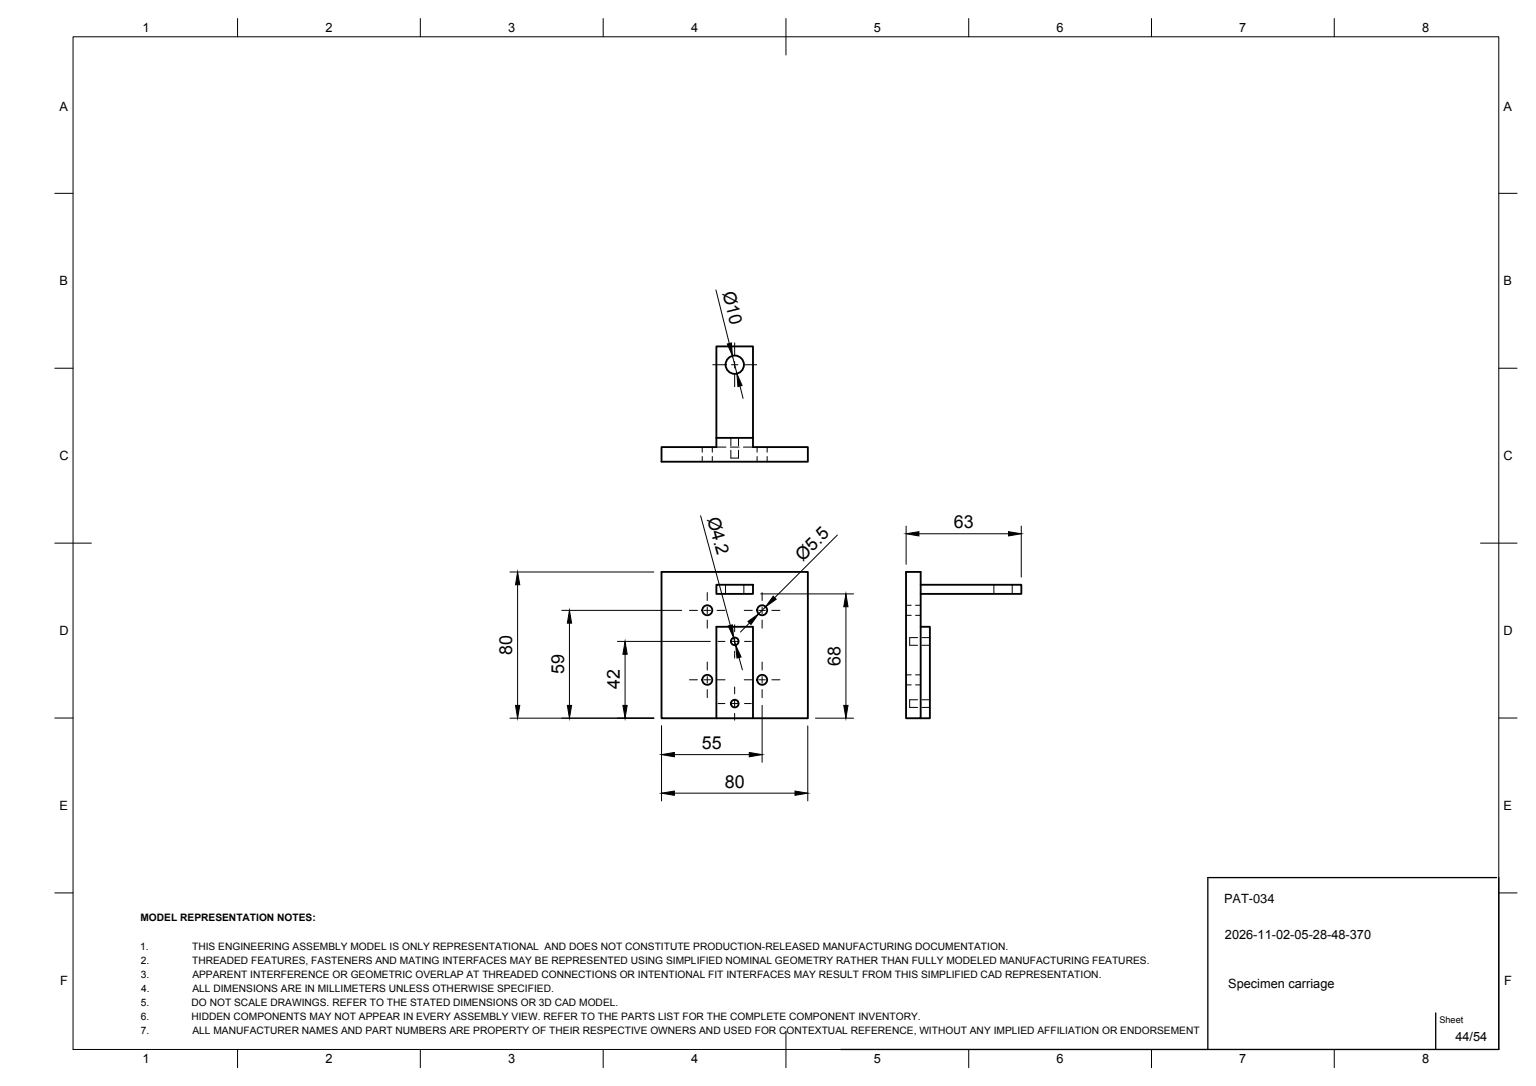
ISO-10303-21;
HEADER;
/* Generated by software containing ST-Developer
 * from STEP Tools, Inc. (www.steptools.com) 
 */

FILE_DESCRIPTION(
/* description */ ('Fatigue rig crank-slider'),
/* implementation_level */ '2;1');

FILE_NAME(
/* name */ 'Specimen carriage.step',
/* time_stamp */ '2026-10-28T03:24:50-07:00',
/* author */ (''),
/* organization */ (''),
/* preprocessor_version */ 'ST-DEVELOPER v20.2',
/* originating_system */ 'Autodesk Translation Framework v15.17.0.0',
/* authorisation */ '');

FILE_SCHEMA (('AUTOMOTIVE_DESIGN { 1 0 10303 214 3 1 1 }'));
ENDSEC;

DATA;
#10=MECHANICAL_DESIGN_GEOMETRIC_PRESENTATION_REPRESENTATION('',(#633),#16911);
#524=SHAPE_REPRESENTATION_RELATIONSHIP('SRR','None',#17168,#574);
#574=ADVANCED_BREP_SHAPE_REPRESENTATION('',(#690),#16897);
#633=STYLED_ITEM('',(#17501),#690);
#690=MANIFOLD_SOLID_BREP('Body1',#8926);
#863=FACE_BOUND('',#2286,.T.);
#864=FACE_BOUND('',#2287,.T.);
#865=FACE_BOUND('',#2291,.T.);
#866=FACE_BOUND('',#2296,.T.);
#867=FACE_BOUND('',#2306,.T.);
#868=FACE_BOUND('',#2307,.T.);
#869=FACE_BOUND('',#2308,.T.);
#870=FACE_BOUND('',#2309,.T.);
#871=FACE_BOUND('',#2310,.T.);
#872=FACE_BOUND('',#2312,.T.);
#873=FACE_BOUND('',#2313,.T.);
#874=FACE_BOUND('',#2314,.T.);
#875=FACE_BOUND('',#2315,.T.);
#1111=PLANE('',#10252);
#1112=PLANE('',#10256);
#1113=PLANE('',#10257);
#1114=PLANE('',#10258);
#1115=PLANE('',#10259);
#1116=PLANE('',#10260);
#1117=PLANE('',#10264);
#1118=PLANE('',#10265);
#1119=PLANE('',#10266);
#1120=PLANE('',#10267);
#1121=PLANE('',#10268);
#1122=PLANE('',#10281);
#1123=PLANE('',#10282);
#1124=PLANE('',#10283);
#1125=PLANE('',#10284);
#1126=PLANE('',#10285);
#1127=PLANE('',#10286);
#1593=FACE_OUTER_BOUND('',#2279,.T.);
#1594=FACE_OUTER_BOUND('',#2280,.T.);
#1595=FACE_OUTER_BOUND('',#2281,.T.);
#1596=FACE_OUTER_BOUND('',#2282,.T.);
#1597=FACE_OUTER_BOUND('',#2283,.T.);
#1598=FACE_OUTER_BOUND('',#2284,.T.);
#1599=FACE_OUTER_BOUND('',#2285,.T.);
#1600=FACE_OUTER_BOUND('',#2288,.T.);
#1601=FACE_OUTER_BOUND('',#2289,.T.);
#1602=FACE_OUTER_BOUND('',#2290,.T.);
#1603=FACE_OUTER_BOUND('',#2292,.T.);
#1604=FACE_OUTER_BOUND('',#2293,.T.);
#1605=FACE_OUTER_BOUND('',#2294,.T.);
#1606=FACE_OUTER_BOUND('',#2295,.T.);
#1607=FACE_OUTER_BOUND('',#2297,.T.);
#1608=FACE_OUTER_BOUND('',#2298,.T.);
#1609=FACE_OUTER_BOUND('',#2299,.T.);
#1610=FACE_OUTER_BOUND('',#2300,.T.);
#1611=FACE_OUTER_BOUND('',#2301,.T.);
#1612=FACE_OUTER_BOUND('',#2302,.T.);
#1613=FACE_OUTER_BOUND('',#2303,.T.);
#1614=FACE_OUTER_BOUND('',#2304,.T.);
#1615=FACE_OUTER_BOUND('',#2305,.T.);
#1616=FACE_OUTER_BOUND('',#2311,.T.);
#2279=EDGE_LOOP('',(#7552,#7553,#7554,#7555));
#2280=EDGE_LOOP('',(#7556));
#2281=EDGE_LOOP('',(#7557,#7558,#7559,#7560));
#2282=EDGE_LOOP('',(#7561));
#2283=EDGE_LOOP('',(#7562,#7563,#7564,#7565));
#2284=EDGE_LOOP('',(#7566,#7567,#7568,#7569));
#2285=EDGE_LOOP('',(#7570,#7571,#7572,#7573));
#2286=EDGE_LOOP('',(#7574));
#2287=EDGE_LOOP('',(#7575));
#2288=EDGE_LOOP('',(#7576,#7577,#7578,#7579));
#2289=EDGE_LOOP('',(#7580,#7581,#7582,#7583));
#2290=EDGE_LOOP('',(#7584,#7585,#7586,#7587));
#2291=EDGE_LOOP('',(#7588));
#2292=EDGE_LOOP('',(#7589,#7590,#7591,#7592));
#2293=EDGE_LOOP('',(#7593,#7594,#7595,#7596));
#2294=EDGE_LOOP('',(#7597,#7598,#7599,#7600));
#2295=EDGE_LOOP('',(#7601,#7602,#7603,#7604));
#2296=EDGE_LOOP('',(#7605));
#2297=EDGE_LOOP('',(#7606,#7607,#7608,#7609));
#2298=EDGE_LOOP('',(#7610,#7611,#7612,#7613));
#2299=EDGE_LOOP('',(#7614,#7615,#7616,#7617));
#2300=EDGE_LOOP('',(#7618,#7619,#7620,#7621));
#2301=EDGE_LOOP('',(#7622,#7623,#7624,#7625));
#2302=EDGE_LOOP('',(#7626,#7627,#7628,#7629));
#2303=EDGE_LOOP('',(#7630,#7631,#7632,#7633,#7634,#7635,#7636,#7637));
#2304=EDGE_LOOP('',(#7638,#7639,#7640,#7641));
#2305=EDGE_LOOP('',(#7642,#7643,#7644,#7645,#7646,#7647,#7648,#7649));
#2306=EDGE_LOOP('',(#7650,#7651,#7652,#7653));
#2307=EDGE_LOOP('',(#7654));
#2308=EDGE_LOOP('',(#7655));
#2309=EDGE_LOOP('',(#7656));
#2310=EDGE_LOOP('',(#7657));
#2311=EDGE_LOOP('',(#7658,#7659,#7660,#7661));
#2312=EDGE_LOOP('',(#7662));
#2313=EDGE_LOOP('',(#7663));
#2314=EDGE_LOOP('',(#7664));
#2315=EDGE_LOOP('',(#7665));
#2863=LINE('',#16027,#3509);
#2864=LINE('',#16034,#3510);
#2865=LINE('',#16040,#3511);
#2866=LINE('',#16042,#3512);
#2867=LINE('',#16044,#3513);
#2868=LINE('',#16045,#3514);
#2869=LINE('',#16049,#3515);
#2870=LINE('',#16051,#3516);
#2871=LINE('',#16053,#3517);
#2872=LINE('',#16054,#3518);
#2873=LINE('',#16056,#3519);
#2874=LINE('',#16057,#3520);
#2875=LINE('',#16059,#3521);
#2876=LINE('',#16064,#3522);
#2877=LINE('',#16069,#3523);
#2878=LINE('',#16071,#3524);
#2879=LINE('',#16073,#3525);
#2880=LINE('',#16074,#3526);
#2881=LINE('',#16077,#3527);
#2882=LINE('',#16079,#3528);
#2883=LINE('',#16080,#3529);
#2884=LINE('',#16083,#3530);
#2885=LINE('',#16085,#3531);
#2886=LINE('',#16086,#3532);
#2887=LINE('',#16088,#3533);
#2888=LINE('',#16090,#3534);
#2889=LINE('',#16095,#3535);
#2890=LINE('',#16101,#3536);
#2891=LINE('',#16107,#3537);
#2892=LINE('',#16113,#3538);
#2893=LINE('',#16118,#3539);
#2894=LINE('',#16120,#3540);
#2895=LINE('',#16122,#3541);
#2896=LINE('',#16123,#3542);
#2897=LINE('',#16126,#3543);
#2898=LINE('',#16128,#3544);
#2899=LINE('',#16129,#3545);
#2900=LINE('',#16132,#3546);
#2901=LINE('',#16133,#3547);
#2902=LINE('',#16135,#3548);
#2903=LINE('',#16136,#3549);
#2904=LINE('',#16138,#3550);
#2905=LINE('',#16139,#3551);
#3509=VECTOR('',#12485,0.210000000000001);
#3510=VECTOR('',#12494,0.210000000000001);
#3511=VECTOR('',#12501,1.);
#3512=VECTOR('',#12502,1.);
#3513=VECTOR('',#12503,1.);
#3514=VECTOR('',#12504,1.);
#3515=VECTOR('',#12507,1.);
#3516=VECTOR('',#12508,1.);
#3517=VECTOR('',#12509,1.);
#3518=VECTOR('',#12510,1.);
#3519=VECTOR('',#12513,1.);
#3520=VECTOR('',#12514,1.);
#3521=VECTOR('',#12517,1.);
#3522=VECTOR('',#12522,0.5);
#3523=VECTOR('',#12527,1.);
#3524=VECTOR('',#12528,1.);
#3525=VECTOR('',#12529,1.);
#3526=VECTOR('',#12530,1.);
#3527=VECTOR('',#12533,1.);
#3528=VECTOR('',#12534,1.);
#3529=VECTOR('',#12535,1.);
#3530=VECTOR('',#12538,1.);
#3531=VECTOR('',#12539,1.);
#3532=VECTOR('',#12540,1.);
#3533=VECTOR('',#12543,1.);
#3534=VECTOR('',#12546,1.);
#3535=VECTOR('',#12551,0.275);
#3536=VECTOR('',#12558,0.275);
#3537=VECTOR('',#12565,0.275);
#3538=VECTOR('',#12572,0.275);
#3539=VECTOR('',#12577,1.);
#3540=VECTOR('',#12578,1.);
#3541=VECTOR('',#12579,1.);
#3542=VECTOR('',#12580,1.);
#3543=VECTOR('',#12583,1.);
#3544=VECTOR('',#12584,1.);
#3545=VECTOR('',#12585,1.);
#3546=VECTOR('',#12588,1.);
#3547=VECTOR('',#12589,1.);
#3548=VECTOR('',#12590,1.);
#3549=VECTOR('',#12591,1.);
#3550=VECTOR('',#12594,1.);
#3551=VECTOR('',#12595,1.);
#4073=CIRCLE('',#10250,0.210000000000001);
#4074=CIRCLE('',#10251,0.210000000000001);
#4075=CIRCLE('',#10254,0.210000000000001);
#4076=CIRCLE('',#10255,0.210000000000001);
#4077=CIRCLE('',#10262,0.5);
#4078=CIRCLE('',#10263,0.5);
#4079=CIRCLE('',#10270,0.275);
#4080=CIRCLE('',#10271,0.275);
#4081=CIRCLE('',#10273,0.275);
#4082=CIRCLE('',#10274,0.275);
#4083=CIRCLE('',#10276,0.275);
#4084=CIRCLE('',#10277,0.275);
#4085=CIRCLE('',#10279,0.275);
#4086=CIRCLE('',#10280,0.275);
#4685=VERTEX_POINT('',#16024);
#4686=VERTEX_POINT('',#16026);
#4687=VERTEX_POINT('',#16031);
#4688=VERTEX_POINT('',#16033);
#4689=VERTEX_POINT('',#16038);
#4690=VERTEX_POINT('',#16039);
#4691=VERTEX_POINT('',#16041);
#4692=VERTEX_POINT('',#16043);
#4693=VERTEX_POINT('',#16047);
#4694=VERTEX_POINT('',#16048);
#4695=VERTEX_POINT('',#16050);
#4696=VERTEX_POINT('',#16052);
#4697=VERTEX_POINT('',#16061);
#4698=VERTEX_POINT('',#16063);
#4699=VERTEX_POINT('',#16067);
#4700=VERTEX_POINT('',#16068);
#4701=VERTEX_POINT('',#16070);
#4702=VERTEX_POINT('',#16072);
#4703=VERTEX_POINT('',#16076);
#4704=VERTEX_POINT('',#16078);
#4705=VERTEX_POINT('',#16082);
#4706=VERTEX_POINT('',#16084);
#4707=VERTEX_POINT('',#16092);
#4708=VERTEX_POINT('',#16094);
#4709=VERTEX_POINT('',#16098);
#4710=VERTEX_POINT('',#16100);
#4711=VERTEX_POINT('',#16104);
#4712=VERTEX_POINT('',#16106);
#4713=VERTEX_POINT('',#16110);
#4714=VERTEX_POINT('',#16112);
#4715=VERTEX_POINT('',#16116);
#4716=VERTEX_POINT('',#16117);
#4717=VERTEX_POINT('',#16119);
#4718=VERTEX_POINT('',#16121);
#4719=VERTEX_POINT('',#16125);
#4720=VERTEX_POINT('',#16127);
#4721=VERTEX_POINT('',#16131);
#4722=VERTEX_POINT('',#16134);
#5674=EDGE_CURVE('',#4685,#4685,#4073,.T.);
#5675=EDGE_CURVE('',#4685,#4686,#2863,.T.);
#5676=EDGE_CURVE('',#4686,#4686,#4074,.T.);
#5677=EDGE_CURVE('',#4687,#4687,#4075,.T.);
#5678=EDGE_CURVE('',#4687,#4688,#2864,.T.);
#5679=EDGE_CURVE('',#4688,#4688,#4076,.T.);
#5680=EDGE_CURVE('',#4689,#4690,#2865,.T.);
#5681=EDGE_CURVE('',#4689,#4691,#2866,.T.);
#5682=EDGE_CURVE('',#4692,#4691,#2867,.T.);
#5683=EDGE_CURVE('',#4690,#4692,#2868,.T.);
#5684=EDGE_CURVE('',#4693,#4694,#2869,.T.);
#5685=EDGE_CURVE('',#4695,#4693,#2870,.T.);
#5686=EDGE_CURVE('',#4696,#4695,#2871,.T.);
#5687=EDGE_CURVE('',#4694,#4696,#2872,.T.);
#5688=EDGE_CURVE('',#4694,#4689,#2873,.T.);
#5689=EDGE_CURVE('',#4691,#4696,#2874,.T.);
#5690=EDGE_CURVE('',#4692,#4695,#2875,.T.);
#5691=EDGE_CURVE('',#4697,#4697,#4077,.T.);
#5692=EDGE_CURVE('',#4697,#4698,#2876,.T.);
#5693=EDGE_CURVE('',#4698,#4698,#4078,.T.);
#5694=EDGE_CURVE('',#4699,#4700,#2877,.T.);
#5695=EDGE_CURVE('',#4699,#4701,#2878,.T.);
#5696=EDGE_CURVE('',#4701,#4702,#2879,.T.);
#5697=EDGE_CURVE('',#4702,#4700,#2880,.T.);
#5698=EDGE_CURVE('',#4703,#4699,#2881,.T.);
#5699=EDGE_CURVE('',#4704,#4703,#2882,.T.);
#5700=EDGE_CURVE('',#4701,#4704,#2883,.T.);
#5701=EDGE_CURVE('',#4700,#4705,#2884,.T.);
#5702=EDGE_CURVE('',#4702,#4706,#2885,.T.);
#5703=EDGE_CURVE('',#4705,#4706,#2886,.T.);
#5704=EDGE_CURVE('',#4706,#4704,#2887,.T.);
#5705=EDGE_CURVE('',#4705,#4703,#2888,.T.);
#5706=EDGE_CURVE('',#4707,#4707,#4079,.T.);
#5707=EDGE_CURVE('',#4707,#4708,#2889,.T.);
#5708=EDGE_CURVE('',#4708,#4708,#4080,.T.);
#5709=EDGE_CURVE('',#4709,#4709,#4081,.T.);
#5710=EDGE_CURVE('',#4709,#4710,#2890,.T.);
#5711=EDGE_CURVE('',#4710,#4710,#4082,.T.);
#5712=EDGE_CURVE('',#4711,#4711,#4083,.T.);
#5713=EDGE_CURVE('',#4711,#4712,#2891,.T.);
#5714=EDGE_CURVE('',#4712,#4712,#4084,.T.);
#5715=EDGE_CURVE('',#4713,#4713,#4085,.T.);
#5716=EDGE_CURVE('',#4713,#4714,#2892,.T.);
#5717=EDGE_CURVE('',#4714,#4714,#4086,.T.);
#5718=EDGE_CURVE('',#4715,#4716,#2893,.T.);
#5719=EDGE_CURVE('',#4716,#4717,#2894,.T.);
#5720=EDGE_CURVE('',#4718,#4717,#2895,.T.);
#5721=EDGE_CURVE('',#4715,#4718,#2896,.T.);
#5722=EDGE_CURVE('',#4719,#4715,#2897,.T.);
#5723=EDGE_CURVE('',#4720,#4718,#2898,.T.);
#5724=EDGE_CURVE('',#4719,#4720,#2899,.T.);
#5725=EDGE_CURVE('',#4721,#4719,#2900,.T.);
#5726=EDGE_CURVE('',#4693,#4720,#2901,.T.);
#5727=EDGE_CURVE('',#4722,#4690,#2902,.T.);
#5728=EDGE_CURVE('',#4721,#4722,#2903,.T.);
#5729=EDGE_CURVE('',#4716,#4721,#2904,.T.);
#5730=EDGE_CURVE('',#4717,#4722,#2905,.T.);
#7552=ORIENTED_EDGE('',*,*,#5674,.F.);
#7553=ORIENTED_EDGE('',*,*,#5675,.T.);
#7554=ORIENTED_EDGE('',*,*,#5676,.F.);
#7555=ORIENTED_EDGE('',*,*,#5675,.F.);
#7556=ORIENTED_EDGE('',*,*,#5674,.T.);
#7557=ORIENTED_EDGE('',*,*,#5677,.F.);
#7558=ORIENTED_EDGE('',*,*,#5678,.T.);
#7559=ORIENTED_EDGE('',*,*,#5679,.F.);
#7560=ORIENTED_EDGE('',*,*,#5678,.F.);
#7561=ORIENTED_EDGE('',*,*,#5677,.T.);
#7562=ORIENTED_EDGE('',*,*,#5680,.F.);
#7563=ORIENTED_EDGE('',*,*,#5681,.T.);
#7564=ORIENTED_EDGE('',*,*,#5682,.F.);
#7565=ORIENTED_EDGE('',*,*,#5683,.F.);
#7566=ORIENTED_EDGE('',*,*,#5684,.F.);
#7567=ORIENTED_EDGE('',*,*,#5685,.F.);
#7568=ORIENTED_EDGE('',*,*,#5686,.F.);
#7569=ORIENTED_EDGE('',*,*,#5687,.F.);
#7570=ORIENTED_EDGE('',*,*,#5688,.F.);
#7571=ORIENTED_EDGE('',*,*,#5687,.T.);
#7572=ORIENTED_EDGE('',*,*,#5689,.F.);
#7573=ORIENTED_EDGE('',*,*,#5681,.F.);
#7574=ORIENTED_EDGE('',*,*,#5676,.T.);
#7575=ORIENTED_EDGE('',*,*,#5679,.T.);
#7576=ORIENTED_EDGE('',*,*,#5689,.T.);
#7577=ORIENTED_EDGE('',*,*,#5686,.T.);
#7578=ORIENTED_EDGE('',*,*,#5690,.F.);
#7579=ORIENTED_EDGE('',*,*,#5682,.T.);
#7580=ORIENTED_EDGE('',*,*,#5691,.F.);
#7581=ORIENTED_EDGE('',*,*,#5692,.T.);
#7582=ORIENTED_EDGE('',*,*,#5693,.F.);
#7583=ORIENTED_EDGE('',*,*,#5692,.F.);
#7584=ORIENTED_EDGE('',*,*,#5694,.F.);
#7585=ORIENTED_EDGE('',*,*,#5695,.T.);
#7586=ORIENTED_EDGE('',*,*,#5696,.T.);
#7587=ORIENTED_EDGE('',*,*,#5697,.T.);
#7588=ORIENTED_EDGE('',*,*,#5691,.T.);
#7589=ORIENTED_EDGE('',*,*,#5698,.F.);
#7590=ORIENTED_EDGE('',*,*,#5699,.F.);
#7591=ORIENTED_EDGE('',*,*,#5700,.F.);
#7592=ORIENTED_EDGE('',*,*,#5695,.F.);
#7593=ORIENTED_EDGE('',*,*,#5701,.F.);
#7594=ORIENTED_EDGE('',*,*,#5697,.F.);
#7595=ORIENTED_EDGE('',*,*,#5702,.T.);
#7596=ORIENTED_EDGE('',*,*,#5703,.F.);
#7597=ORIENTED_EDGE('',*,*,#5696,.F.);
#7598=ORIENTED_EDGE('',*,*,#5700,.T.);
#7599=ORIENTED_EDGE('',*,*,#5704,.F.);
#7600=ORIENTED_EDGE('',*,*,#5702,.F.);
#7601=ORIENTED_EDGE('',*,*,#5705,.F.);
#7602=ORIENTED_EDGE('',*,*,#5703,.T.);
#7603=ORIENTED_EDGE('',*,*,#5704,.T.);
#7604=ORIENTED_EDGE('',*,*,#5699,.T.);
#7605=ORIENTED_EDGE('',*,*,#5693,.T.);
#7606=ORIENTED_EDGE('',*,*,#5706,.F.);
#7607=ORIENTED_EDGE('',*,*,#5707,.T.);
#7608=ORIENTED_EDGE('',*,*,#5708,.F.);
#7609=ORIENTED_EDGE('',*,*,#5707,.F.);
#7610=ORIENTED_EDGE('',*,*,#5709,.F.);
#7611=ORIENTED_EDGE('',*,*,#5710,.T.);
#7612=ORIENTED_EDGE('',*,*,#5711,.F.);
#7613=ORIENTED_EDGE('',*,*,#5710,.F.);
#7614=ORIENTED_EDGE('',*,*,#5712,.F.);
#7615=ORIENTED_EDGE('',*,*,#5713,.T.);
#7616=ORIENTED_EDGE('',*,*,#5714,.F.);
#7617=ORIENTED_EDGE('',*,*,#5713,.F.);
#7618=ORIENTED_EDGE('',*,*,#5715,.F.);
#7619=ORIENTED_EDGE('',*,*,#5716,.T.);
#7620=ORIENTED_EDGE('',*,*,#5717,.F.);
#7621=ORIENTED_EDGE('',*,*,#5716,.F.);
#7622=ORIENTED_EDGE('',*,*,#5718,.T.);
#7623=ORIENTED_EDGE('',*,*,#5719,.T.);
#7624=ORIENTED_EDGE('',*,*,#5720,.F.);
#7625=ORIENTED_EDGE('',*,*,#5721,.F.);
#7626=ORIENTED_EDGE('',*,*,#5722,.T.);
#7627=ORIENTED_EDGE('',*,*,#5721,.T.);
#7628=ORIENTED_EDGE('',*,*,#5723,.F.);
#7629=ORIENTED_EDGE('',*,*,#5724,.F.);
#7630=ORIENTED_EDGE('',*,*,#5725,.T.);
#7631=ORIENTED_EDGE('',*,*,#5724,.T.);
#7632=ORIENTED_EDGE('',*,*,#5726,.F.);
#7633=ORIENTED_EDGE('',*,*,#5684,.T.);
#7634=ORIENTED_EDGE('',*,*,#5688,.T.);
#7635=ORIENTED_EDGE('',*,*,#5680,.T.);
#7636=ORIENTED_EDGE('',*,*,#5727,.F.);
#7637=ORIENTED_EDGE('',*,*,#5728,.F.);
#7638=ORIENTED_EDGE('',*,*,#5729,.T.);
#7639=ORIENTED_EDGE('',*,*,#5728,.T.);
#7640=ORIENTED_EDGE('',*,*,#5730,.F.);
#7641=ORIENTED_EDGE('',*,*,#5719,.F.);
#7642=ORIENTED_EDGE('',*,*,#5685,.T.);
#7643=ORIENTED_EDGE('',*,*,#5726,.T.);
#7644=ORIENTED_EDGE('',*,*,#5723,.T.);
#7645=ORIENTED_EDGE('',*,*,#5720,.T.);
#7646=ORIENTED_EDGE('',*,*,#5730,.T.);
#7647=ORIENTED_EDGE('',*,*,#5727,.T.);
#7648=ORIENTED_EDGE('',*,*,#5683,.T.);
#7649=ORIENTED_EDGE('',*,*,#5690,.T.);
#7650=ORIENTED_EDGE('',*,*,#5698,.T.);
#7651=ORIENTED_EDGE('',*,*,#5694,.T.);
#7652=ORIENTED_EDGE('',*,*,#5701,.T.);
#7653=ORIENTED_EDGE('',*,*,#5705,.T.);
#7654=ORIENTED_EDGE('',*,*,#5708,.T.);
#7655=ORIENTED_EDGE('',*,*,#5711,.T.);
#7656=ORIENTED_EDGE('',*,*,#5714,.T.);
#7657=ORIENTED_EDGE('',*,*,#5717,.T.);
#7658=ORIENTED_EDGE('',*,*,#5729,.F.);
#7659=ORIENTED_EDGE('',*,*,#5718,.F.);
#7660=ORIENTED_EDGE('',*,*,#5722,.F.);
#7661=ORIENTED_EDGE('',*,*,#5725,.F.);
#7662=ORIENTED_EDGE('',*,*,#5706,.T.);
#7663=ORIENTED_EDGE('',*,*,#5709,.T.);
#7664=ORIENTED_EDGE('',*,*,#5712,.T.);
#7665=ORIENTED_EDGE('',*,*,#5715,.T.);
#8325=CYLINDRICAL_SURFACE('',#10249,0.210000000000001);
#8326=CYLINDRICAL_SURFACE('',#10253,0.210000000000001);
#8327=CYLINDRICAL_SURFACE('',#10261,0.5);
#8328=CYLINDRICAL_SURFACE('',#10269,0.275);
#8329=CYLINDRICAL_SURFACE('',#10272,0.275);
#8330=CYLINDRICAL_SURFACE('',#10275,0.275);
#8331=CYLINDRICAL_SURFACE('',#10278,0.275);
#8731=ADVANCED_FACE('',(#1593),#8325,.F.);
#8732=ADVANCED_FACE('',(#1594),#1111,.T.);
#8733=ADVANCED_FACE('',(#1595),#8326,.F.);
#8734=ADVANCED_FACE('',(#1596),#1112,.T.);
#8735=ADVANCED_FACE('',(#1597),#1113,.T.);
#8736=ADVANCED_FACE('',(#1598),#1114,.T.);
#8737=ADVANCED_FACE('',(#1599,#863,#864),#1115,.T.);
#8738=ADVANCED_FACE('',(#1600),#1116,.T.);
#8739=ADVANCED_FACE('',(#1601),#8327,.F.);
#8740=ADVANCED_FACE('',(#1602,#865),#1117,.F.);
#8741=ADVANCED_FACE('',(#1603),#1118,.T.);
#8742=ADVANCED_FACE('',(#1604),#1119,.T.);
#8743=ADVANCED_FACE('',(#1605),#1120,.T.);
#8744=ADVANCED_FACE('',(#1606,#866),#1121,.T.);
#8745=ADVANCED_FACE('',(#1607),#8328,.F.);
#8746=ADVANCED_FACE('',(#1608),#8329,.F.);
#8747=ADVANCED_FACE('',(#1609),#8330,.F.);
#8748=ADVANCED_FACE('',(#1610),#8331,.F.);
#8749=ADVANCED_FACE('',(#1611),#1122,.T.);
#8750=ADVANCED_FACE('',(#1612),#1123,.T.);
#8751=ADVANCED_FACE('',(#1613),#1124,.T.);
#8752=ADVANCED_FACE('',(#1614),#1125,.T.);
#8753=ADVANCED_FACE('',(#1615,#867,#868,#869,#870,#871),#1126,.T.);
#8754=ADVANCED_FACE('',(#1616,#872,#873,#874,#875),#1127,.F.);
#8926=CLOSED_SHELL('',(#8731,#8732,#8733,#8734,#8735,#8736,#8737,#8738,
#8739,#8740,#8741,#8742,#8743,#8744,#8745,#8746,#8747,#8748,#8749,#8750,
#8751,#8752,#8753,#8754));
#10248=AXIS2_PLACEMENT_3D('',#16022,#12479,#12480);
#10249=AXIS2_PLACEMENT_3D('',#16023,#12481,#12482);
#10250=AXIS2_PLACEMENT_3D('',#16025,#12483,#12484);
#10251=AXIS2_PLACEMENT_3D('',#16028,#12486,#12487);
#10252=AXIS2_PLACEMENT_3D('',#16029,#12488,#12489);
#10253=AXIS2_PLACEMENT_3D('',#16030,#12490,#12491);
#10254=AXIS2_PLACEMENT_3D('',#16032,#12492,#12493);
#10255=AXIS2_PLACEMENT_3D('',#16035,#12495,#12496);
#10256=AXIS2_PLACEMENT_3D('',#16036,#12497,#12498);
#10257=AXIS2_PLACEMENT_3D('',#16037,#12499,#12500);
#10258=AXIS2_PLACEMENT_3D('',#16046,#12505,#12506);
#10259=AXIS2_PLACEMENT_3D('',#16055,#12511,#12512);
#10260=AXIS2_PLACEMENT_3D('',#16058,#12515,#12516);
#10261=AXIS2_PLACEMENT_3D('',#16060,#12518,#12519);
#10262=AXIS2_PLACEMENT_3D('',#16062,#12520,#12521);
#10263=AXIS2_PLACEMENT_3D('',#16065,#12523,#12524);
#10264=AXIS2_PLACEMENT_3D('',#16066,#12525,#12526);
#10265=AXIS2_PLACEMENT_3D('',#16075,#12531,#12532);
#10266=AXIS2_PLACEMENT_3D('',#16081,#12536,#12537);
#10267=AXIS2_PLACEMENT_3D('',#16087,#12541,#12542);
#10268=AXIS2_PLACEMENT_3D('',#16089,#12544,#12545);
#10269=AXIS2_PLACEMENT_3D('',#16091,#12547,#12548);
#10270=AXIS2_PLACEMENT_3D('',#16093,#12549,#12550);
#10271=AXIS2_PLACEMENT_3D('',#16096,#12552,#12553);
#10272=AXIS2_PLACEMENT_3D('',#16097,#12554,#12555);
#10273=AXIS2_PLACEMENT_3D('',#16099,#12556,#12557);
#10274=AXIS2_PLACEMENT_3D('',#16102,#12559,#12560);
#10275=AXIS2_PLACEMENT_3D('',#16103,#12561,#12562);
#10276=AXIS2_PLACEMENT_3D('',#16105,#12563,#12564);
#10277=AXIS2_PLACEMENT_3D('',#16108,#12566,#12567);
#10278=AXIS2_PLACEMENT_3D('',#16109,#12568,#12569);
#10279=AXIS2_PLACEMENT_3D('',#16111,#12570,#12571);
#10280=AXIS2_PLACEMENT_3D('',#16114,#12573,#12574);
#10281=AXIS2_PLACEMENT_3D('',#16115,#12575,#12576);
#10282=AXIS2_PLACEMENT_3D('',#16124,#12581,#12582);
#10283=AXIS2_PLACEMENT_3D('',#16130,#12586,#12587);
#10284=AXIS2_PLACEMENT_3D('',#16137,#12592,#12593);
#10285=AXIS2_PLACEMENT_3D('',#16140,#12596,#12597);
#10286=AXIS2_PLACEMENT_3D('',#16141,#12598,#12599);
#12479=DIRECTION('axis',(0.,0.,1.));
#12480=DIRECTION('refdir',(1.,0.,0.));
#12481=DIRECTION('center_axis',(0.,0.,1.));
#12482=DIRECTION('ref_axis',(1.,0.,0.));
#12483=DIRECTION('center_axis',(0.,0.,1.));
#12484=DIRECTION('ref_axis',(1.,0.,0.));
#12485=DIRECTION('',(0.,0.,1.));
#12486=DIRECTION('center_axis',(0.,0.,-1.));
#12487=DIRECTION('ref_axis',(1.,0.,0.));
#12488=DIRECTION('center_axis',(0.,0.,1.));
#12489=DIRECTION('ref_axis',(1.,0.,0.));
#12490=DIRECTION('center_axis',(0.,0.,1.));
#12491=DIRECTION('ref_axis',(1.,0.,0.));
#12492=DIRECTION('center_axis',(0.,0.,1.));
#12493=DIRECTION('ref_axis',(1.,0.,0.));
#12494=DIRECTION('',(0.,0.,1.));
#12495=DIRECTION('center_axis',(0.,0.,-1.));
#12496=DIRECTION('ref_axis',(1.,0.,0.));
#12497=DIRECTION('center_axis',(0.,0.,1.));
#12498=DIRECTION('ref_axis',(1.,0.,0.));
#12499=DIRECTION('center_axis',(-1.,0.,0.));
#12500=DIRECTION('ref_axis',(0.,0.,1.));
#12501=DIRECTION('',(0.,0.,-1.));
#12502=DIRECTION('',(0.,1.,0.));
#12503=DIRECTION('',(0.,0.,1.));
#12504=DIRECTION('',(0.,1.,0.));
#12505=DIRECTION('center_axis',(1.,0.,0.));
#12506=DIRECTION('ref_axis',(0.,0.,-1.));
#12507=DIRECTION('',(0.,0.,1.));
#12508=DIRECTION('',(0.,-1.,0.));
#12509=DIRECTION('',(0.,0.,-1.));
#12510=DIRECTION('',(0.,1.,0.));
#12511=DIRECTION('center_axis',(0.,0.,1.));
#12512=DIRECTION('ref_axis',(1.,0.,0.));
#12513=DIRECTION('',(-1.,0.,0.));
#12514=DIRECTION('',(1.,0.,0.));
#12515=DIRECTION('center_axis',(0.,1.,0.));
#12516=DIRECTION('ref_axis',(0.,0.,1.));
#12517=DIRECTION('',(1.,0.,0.));
#12518=DIRECTION('center_axis',(0.,1.,0.));
#12519=DIRECTION('ref_axis',(1.,0.,0.));
#12520=DIRECTION('center_axis',(0.,1.,0.));
#12521=DIRECTION('ref_axis',(1.,0.,0.));
#12522=DIRECTION('',(0.,1.,0.));
#12523=DIRECTION('center_axis',(0.,-1.,0.));
#12524=DIRECTION('ref_axis',(1.,0.,0.));
#12525=DIRECTION('center_axis',(0.,1.,0.));
#12526=DIRECTION('ref_axis',(1.,0.,0.));
#12527=DIRECTION('',(-1.,0.,0.));
#12528=DIRECTION('',(0.,0.,1.));
#12529=DIRECTION('',(-1.,0.,0.));
#12530=DIRECTION('',(0.,0.,-1.));
#12531=DIRECTION('center_axis',(1.,0.,0.));
#12532=DIRECTION('ref_axis',(0.,0.,-1.));
#12533=DIRECTION('',(0.,-1.,0.));
#12534=DIRECTION('',(0.,0.,-1.));
#12535=DIRECTION('',(0.,1.,0.));
#12536=DIRECTION('center_axis',(-1.,0.,0.));
#12537=DIRECTION('ref_axis',(0.,0.,1.));
#12538=DIRECTION('',(0.,1.,0.));
#12539=DIRECTION('',(0.,1.,0.));
#12540=DIRECTION('',(0.,0.,1.));
#12541=DIRECTION('center_axis',(0.,0.,1.));
#12542=DIRECTION('ref_axis',(1.,0.,0.));
#12543=DIRECTION('',(1.,0.,0.));
#12544=DIRECTION('center_axis',(0.,1.,0.));
#12545=DIRECTION('ref_axis',(0.,0.,1.));
#12546=DIRECTION('',(1.,0.,0.));
#12547=DIRECTION('center_axis',(0.,0.,1.));
#12548=DIRECTION('ref_axis',(1.,0.,0.));
#12549=DIRECTION('center_axis',(0.,0.,1.));
#12550=DIRECTION('ref_axis',(1.,0.,0.));
#12551=DIRECTION('',(0.,0.,1.));
#12552=DIRECTION('center_axis',(0.,0.,-1.));
#12553=DIRECTION('ref_axis',(1.,0.,0.));
#12554=DIRECTION('center_axis',(0.,0.,1.));
#12555=DIRECTION('ref_axis',(1.,0.,0.));
#12556=DIRECTION('center_axis',(0.,0.,1.));
#12557=DIRECTION('ref_axis',(1.,0.,0.));
#12558=DIRECTION('',(0.,0.,1.));
#12559=DIRECTION('center_axis',(0.,0.,-1.));
#12560=DIRECTION('ref_axis',(1.,0.,0.));
#12561=DIRECTION('center_axis',(0.,0.,1.));
#12562=DIRECTION('ref_axis',(1.,0.,0.));
#12563=DIRECTION('center_axis',(0.,0.,1.));
#12564=DIRECTION('ref_axis',(1.,0.,0.));
#12565=DIRECTION('',(0.,0.,1.));
#12566=DIRECTION('center_axis',(0.,0.,-1.));
#12567=DIRECTION('ref_axis',(1.,0.,0.));
#12568=DIRECTION('center_axis',(0.,0.,1.));
#12569=DIRECTION('ref_axis',(1.,0.,0.));
#12570=DIRECTION('center_axis',(0.,0.,1.));
#12571=DIRECTION('ref_axis',(1.,0.,0.));
#12572=DIRECTION('',(0.,0.,1.));
#12573=DIRECTION('center_axis',(0.,0.,-1.));
#12574=DIRECTION('ref_axis',(1.,0.,0.));
#12575=DIRECTION('center_axis',(0.,1.,0.));
#12576=DIRECTION('ref_axis',(-1.,0.,0.));
#12577=DIRECTION('',(-1.,0.,0.));
#12578=DIRECTION('',(0.,0.,1.));
#12579=DIRECTION('',(-1.,0.,0.));
#12580=DIRECTION('',(0.,0.,1.));
#12581=DIRECTION('center_axis',(1.,0.,0.));
#12582=DIRECTION('ref_axis',(0.,1.,0.));
#12583=DIRECTION('',(0.,1.,0.));
#12584=DIRECTION('',(0.,1.,0.));
#12585=DIRECTION('',(0.,0.,1.));
#12586=DIRECTION('center_axis',(0.,-1.,0.));
#12587=DIRECTION('ref_axis',(1.,0.,0.));
#12588=DIRECTION('',(1.,0.,0.));
#12589=DIRECTION('',(1.,0.,0.));
#12590=DIRECTION('',(1.,0.,0.));
#12591=DIRECTION('',(0.,0.,1.));
#12592=DIRECTION('center_axis',(-1.,0.,0.));
#12593=DIRECTION('ref_axis',(0.,-1.,0.));
#12594=DIRECTION('',(0.,-1.,0.));
#12595=DIRECTION('',(0.,-1.,0.));
#12596=DIRECTION('center_axis',(0.,0.,1.));
#12597=DIRECTION('ref_axis',(1.,0.,0.));
#12598=DIRECTION('center_axis',(0.,0.,1.));
#12599=DIRECTION('ref_axis',(1.,0.,0.));
#16022=CARTESIAN_POINT('',(0.,0.,0.));
#16023=CARTESIAN_POINT('Origin',(11.,-3.2,6.9));
#16024=CARTESIAN_POINT('',(10.79,-3.2,6.9));
#16025=CARTESIAN_POINT('Origin',(11.,-3.2,6.9));
#16026=CARTESIAN_POINT('',(10.79,-3.2,8.));
#16027=CARTESIAN_POINT('',(10.79,-3.2,6.9));
#16028=CARTESIAN_POINT('Origin',(11.,-3.2,8.));
#16029=CARTESIAN_POINT('Origin',(11.,-3.2,6.9));
#16030=CARTESIAN_POINT('Origin',(11.,0.2,6.9));
#16031=CARTESIAN_POINT('',(10.79,0.2,6.9));
#16032=CARTESIAN_POINT('Origin',(11.,0.2,6.9));
#16033=CARTESIAN_POINT('',(10.79,0.2,8.));
#16034=CARTESIAN_POINT('',(10.79,0.2,6.9));
#16035=CARTESIAN_POINT('Origin',(11.,0.2,8.));
#16036=CARTESIAN_POINT('Origin',(11.,0.2,6.9));
#16037=CARTESIAN_POINT('Origin',(10.,-4.,7.5));
#16038=CARTESIAN_POINT('',(10.,-4.,8.));
#16039=CARTESIAN_POINT('',(10.,-4.,7.5));
#16040=CARTESIAN_POINT('',(10.,-4.,8.));
#16041=CARTESIAN_POINT('',(10.,1.,8.));
#16042=CARTESIAN_POINT('',(10.,-4.,8.));
#16043=CARTESIAN_POINT('',(10.,1.,7.5));
#16044=CARTESIAN_POINT('',(10.,1.,8.));
#16045=CARTESIAN_POINT('',(10.,-2.,7.5));
#16046=CARTESIAN_POINT('Origin',(12.,-4.,8.));
#16047=CARTESIAN_POINT('',(12.,-4.,7.5));
#16048=CARTESIAN_POINT('',(12.,-4.,8.));
#16049=CARTESIAN_POINT('',(12.,-4.,7.5));
#16050=CARTESIAN_POINT('',(12.,1.,7.5));
#16051=CARTESIAN_POINT('',(12.,-2.,7.5));
#16052=CARTESIAN_POINT('',(12.,1.,8.));
#16053=CARTESIAN_POINT('',(12.,1.,7.5));
#16054=CARTESIAN_POINT('',(12.,-4.,8.));
#16055=CARTESIAN_POINT('Origin',(10.,-4.,8.));
#16056=CARTESIAN_POINT('',(12.,-4.,8.));
#16057=CARTESIAN_POINT('',(12.,1.,8.));
#16058=CARTESIAN_POINT('Origin',(11.,1.,7.75));
#16059=CARTESIAN_POINT('',(11.,1.,7.5));
#16060=CARTESIAN_POINT('Origin',(11.,2.7,12.));
#16061=CARTESIAN_POINT('',(10.5,2.8,12.));
#16062=CARTESIAN_POINT('Origin',(11.,2.8,12.));
#16063=CARTESIAN_POINT('',(10.5,3.3,12.));
#16064=CARTESIAN_POINT('',(10.5,2.7,12.));
#16065=CARTESIAN_POINT('Origin',(11.,3.3,12.));
#16066=CARTESIAN_POINT('Origin',(11.,2.8,10.15));
#16067=CARTESIAN_POINT('',(12.,2.8,7.5));
#16068=CARTESIAN_POINT('',(10.,2.8,7.5));
#16069=CARTESIAN_POINT('',(11.,2.8,7.5));
#16070=CARTESIAN_POINT('',(12.,2.8,13.));
#16071=CARTESIAN_POINT('',(12.,2.8,7.3));
#16072=CARTESIAN_POINT('',(10.,2.8,13.));
#16073=CARTESIAN_POINT('',(12.,2.8,13.));
#16074=CARTESIAN_POINT('',(10.,2.8,13.));
#16075=CARTESIAN_POINT('Origin',(12.,2.8,13.));
#16076=CARTESIAN_POINT('',(12.,3.3,7.5));
#16077=CARTESIAN_POINT('',(12.,1.4,7.5));
#16078=CARTESIAN_POINT('',(12.,3.3,13.));
#16079=CARTESIAN_POINT('',(12.,3.3,7.3));
#16080=CARTESIAN_POINT('',(12.,2.8,13.));
#16081=CARTESIAN_POINT('Origin',(10.,2.8,7.3));
#16082=CARTESIAN_POINT('',(10.,3.3,7.5));
#16083=CARTESIAN_POINT('',(10.,1.4,7.5));
#16084=CARTESIAN_POINT('',(10.,3.3,13.));
#16085=CARTESIAN_POINT('',(10.,2.8,13.));
#16086=CARTESIAN_POINT('',(10.,3.3,13.));
#16087=CARTESIAN_POINT('Origin',(10.,2.8,13.));
#16088=CARTESIAN_POINT('',(12.,3.3,13.));
#16089=CARTESIAN_POINT('Origin',(11.,3.3,10.15));
#16090=CARTESIAN_POINT('',(11.,3.3,7.5));
#16091=CARTESIAN_POINT('Origin',(12.5,-1.9,6.6));
#16092=CARTESIAN_POINT('',(12.225,-1.9,6.7));
#16093=CARTESIAN_POINT('Origin',(12.5,-1.9,6.7));
#16094=CARTESIAN_POINT('',(12.225,-1.9,7.5));
#16095=CARTESIAN_POINT('',(12.225,-1.9,6.6));
#16096=CARTESIAN_POINT('Origin',(12.5,-1.9,7.5));
#16097=CARTESIAN_POINT('Origin',(9.5,1.9,6.6));
#16098=CARTESIAN_POINT('',(9.225,1.9,6.7));
#16099=CARTESIAN_POINT('Origin',(9.5,1.9,6.7));
#16100=CARTESIAN_POINT('',(9.225,1.9,7.5));
#16101=CARTESIAN_POINT('',(9.225,1.9,6.6));
#16102=CARTESIAN_POINT('Origin',(9.5,1.9,7.5));
#16103=CARTESIAN_POINT('Origin',(9.5,-1.9,6.6));
#16104=CARTESIAN_POINT('',(9.225,-1.9,6.7));
#16105=CARTESIAN_POINT('Origin',(9.5,-1.9,6.7));
#16106=CARTESIAN_POINT('',(9.225,-1.9,7.5));
#16107=CARTESIAN_POINT('',(9.225,-1.9,6.6));
#16108=CARTESIAN_POINT('Origin',(9.5,-1.9,7.5));
#16109=CARTESIAN_POINT('Origin',(12.5,1.9,6.6));
#16110=CARTESIAN_POINT('',(12.225,1.9,6.7));
#16111=CARTESIAN_POINT('Origin',(12.5,1.9,6.7));
#16112=CARTESIAN_POINT('',(12.225,1.9,7.5));
#16113=CARTESIAN_POINT('',(12.225,1.9,6.6));
#16114=CARTESIAN_POINT('Origin',(12.5,1.9,7.5));
#16115=CARTESIAN_POINT('Origin',(15.,4.,6.7));
#16116=CARTESIAN_POINT('',(15.,4.,6.7));
#16117=CARTESIAN_POINT('',(7.,4.,6.7));
#16118=CARTESIAN_POINT('',(15.,4.,6.7));
#16119=CARTESIAN_POINT('',(7.,4.,7.5));
#16120=CARTESIAN_POINT('',(7.,4.,6.7));
#16121=CARTESIAN_POINT('',(15.,4.,7.5));
#16122=CARTESIAN_POINT('',(15.,4.,7.5));
#16123=CARTESIAN_POINT('',(15.,4.,6.7));
#16124=CARTESIAN_POINT('Origin',(15.,-4.,6.7));
#16125=CARTESIAN_POINT('',(15.,-4.,6.7));
#16126=CARTESIAN_POINT('',(15.,-4.,6.7));
#16127=CARTESIAN_POINT('',(15.,-4.,7.5));
#16128=CARTESIAN_POINT('',(15.,-4.,7.5));
#16129=CARTESIAN_POINT('',(15.,-4.,6.7));
#16130=CARTESIAN_POINT('Origin',(7.,-4.,6.7));
#16131=CARTESIAN_POINT('',(7.,-4.,6.7));
#16132=CARTESIAN_POINT('',(7.,-4.,6.7));
#16133=CARTESIAN_POINT('',(7.,-4.,7.5));
#16134=CARTESIAN_POINT('',(7.,-4.,7.5));
#16135=CARTESIAN_POINT('',(7.,-4.,7.5));
#16136=CARTESIAN_POINT('',(7.,-4.,6.7));
#16137=CARTESIAN_POINT('Origin',(7.,4.,6.7));
#16138=CARTESIAN_POINT('',(7.,4.,6.7));
#16139=CARTESIAN_POINT('',(7.,4.,7.5));
#16140=CARTESIAN_POINT('Origin',(11.,0.,7.5));
#16141=CARTESIAN_POINT('Origin',(11.,0.,6.7));
#16838=UNCERTAINTY_MEASURE_WITH_UNIT(LENGTH_MEASURE(0.001),#16912,
'DISTANCE_ACCURACY_VALUE',
'Maximum model space distance between geometric entities at asserted c
onnectivities');
#16852=UNCERTAINTY_MEASURE_WITH_UNIT(LENGTH_MEASURE(0.001),#16912,
'DISTANCE_ACCURACY_VALUE',
'Maximum model space distance between geometric entities at asserted c
onnectivities');
#16897=(
GEOMETRIC_REPRESENTATION_CONTEXT(3)
GLOBAL_UNCERTAINTY_ASSIGNED_CONTEXT((#16838))
GLOBAL_UNIT_ASSIGNED_CONTEXT((#16912,#16914,#16915))
REPRESENTATION_CONTEXT('','3D')
);
#16911=(
GEOMETRIC_REPRESENTATION_CONTEXT(3)
GLOBAL_UNCERTAINTY_ASSIGNED_CONTEXT((#16852))
GLOBAL_UNIT_ASSIGNED_CONTEXT((#16912,#16914,#16915))
REPRESENTATION_CONTEXT('','3D')
);
#16912=(
LENGTH_UNIT()
NAMED_UNIT(*)
SI_UNIT(.CENTI.,.METRE.)
);
#16914=(
NAMED_UNIT(*)
PLANE_ANGLE_UNIT()
SI_UNIT($,.RADIAN.)
);
#16915=(
NAMED_UNIT(*)
SI_UNIT($,.STERADIAN.)
SOLID_ANGLE_UNIT()
);
#16960=SHAPE_DEFINITION_REPRESENTATION(#17032,#17168);
#17032=PRODUCT_DEFINITION_SHAPE('',$,#17227);
#17168=SHAPE_REPRESENTATION('',(#10248),#16897);
#17182=PRODUCT_DEFINITION_CONTEXT('part definition',#17358,'design');
#17227=PRODUCT_DEFINITION('Specimen carriage','Specimen carriage',#17285,
#17182);
#17285=PRODUCT_DEFINITION_FORMATION('',$,#17404);
#17358=APPLICATION_CONTEXT(
'Core Data for Automotive Mechanical Design Process');
#17359=PRODUCT_CONTEXT('part definition',#17358,'mechanical');
#17404=PRODUCT('Specimen carriage','Specimen carriage',
'Specimen carriage',(#17359));
#17495=COLOUR_RGB('Off White',0.89,0.88,0.83);
#17496=FILL_AREA_STYLE_COLOUR('',#17495);
#17497=FILL_AREA_STYLE('',(#17496));
#17498=SURFACE_STYLE_FILL_AREA(#17497);
#17499=SURFACE_SIDE_STYLE('',(#17498));
#17500=SURFACE_STYLE_USAGE(.BOTH.,#17499);
#17501=PRESENTATION_STYLE_ASSIGNMENT((#17500));
ENDSEC;
END-ISO-10303-21;
